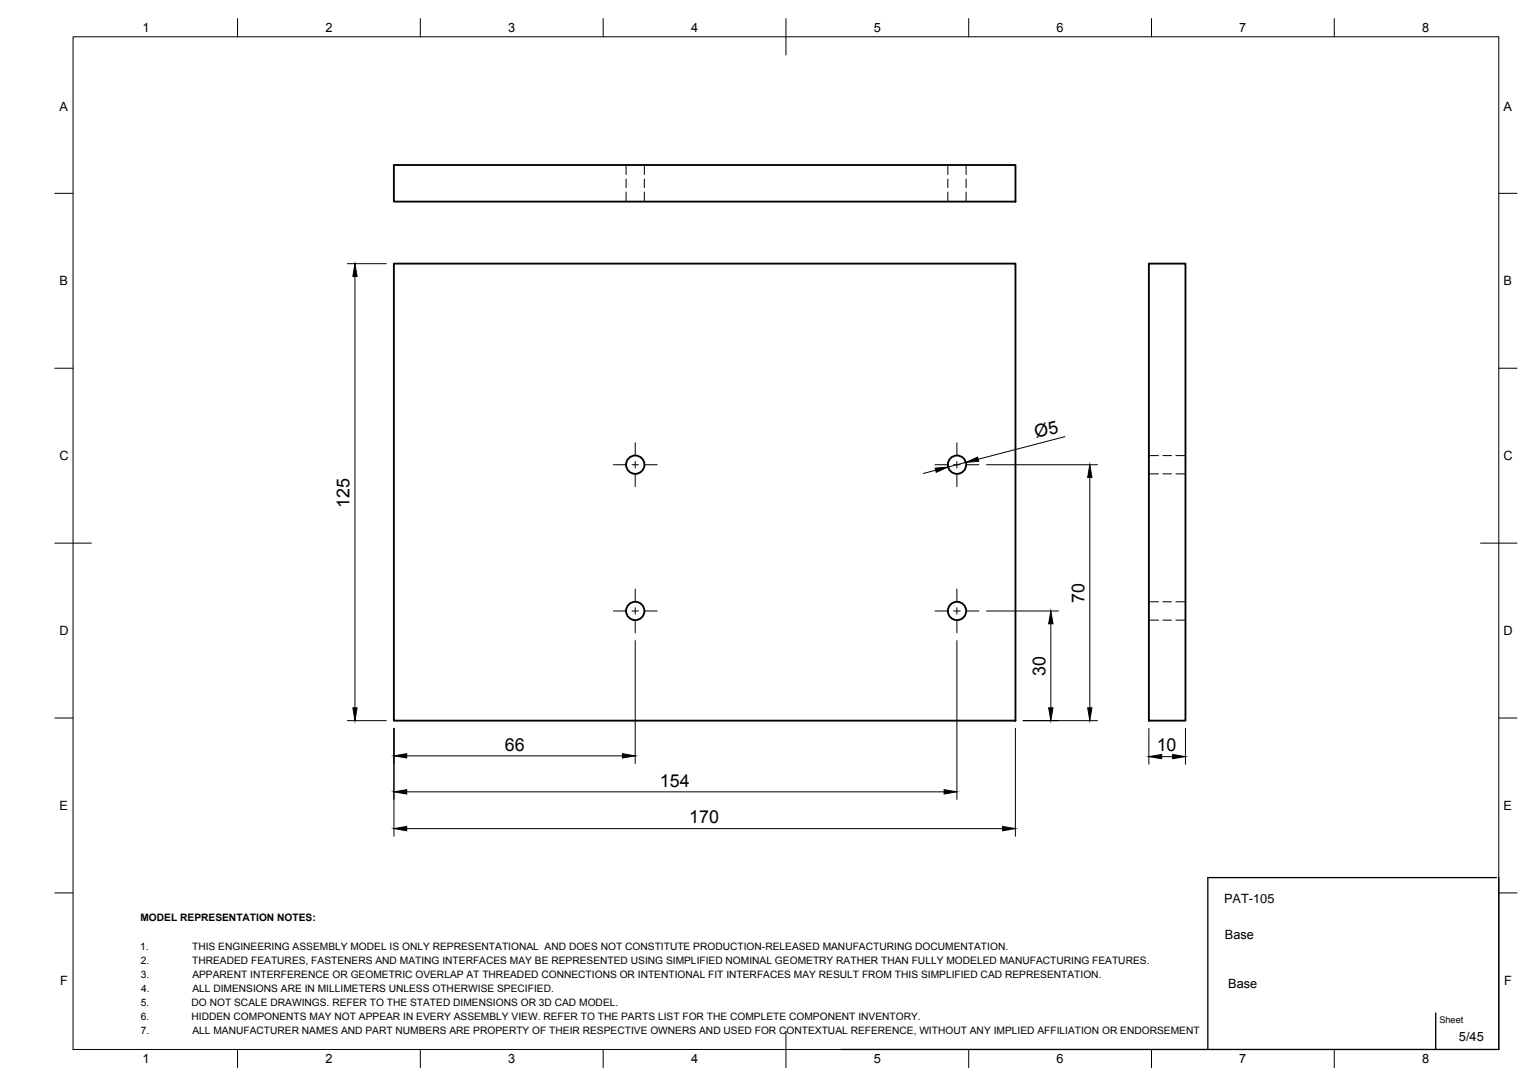
ISO-10303-21;
HEADER;
/* Generated by software containing ST-Developer
 * from STEP Tools, Inc. (www.steptools.com) 
 */

FILE_DESCRIPTION(
/* description */ ('Torque wrench calibration arm'),
/* implementation_level */ '2;1');

FILE_NAME(
/* name */ 'Base.step',
/* time_stamp */ '2026-10-28T03:24:52-07:00',
/* author */ (''),
/* organization */ (''),
/* preprocessor_version */ 'ST-DEVELOPER v20.2',
/* originating_system */ 'Autodesk Translation Framework v15.17.0.0',
/* authorisation */ '');

FILE_SCHEMA (('AUTOMOTIVE_DESIGN { 1 0 10303 214 3 1 1 }'));
ENDSEC;

DATA;
#10=MECHANICAL_DESIGN_GEOMETRIC_PRESENTATION_REPRESENTATION('',(#426),#12783);
#352=SHAPE_REPRESENTATION_RELATIONSHIP('SRR','None',#12933,#389);
#389=ADVANCED_BREP_SHAPE_REPRESENTATION('',(#480),#12742);
#426=STYLED_ITEM('',(#13191),#480);
#480=MANIFOLD_SOLID_BREP('Body1',#6495);
#531=FACE_BOUND('',#1279,.T.);
#532=FACE_BOUND('',#1280,.T.);
#533=FACE_BOUND('',#1281,.T.);
#534=FACE_BOUND('',#1282,.T.);
#535=FACE_BOUND('',#1284,.T.);
#536=FACE_BOUND('',#1285,.T.);
#537=FACE_BOUND('',#1286,.T.);
#538=FACE_BOUND('',#1287,.T.);
#652=PLANE('',#6975);
#653=PLANE('',#6976);
#654=PLANE('',#6977);
#655=PLANE('',#6978);
#656=PLANE('',#6979);
#657=PLANE('',#6980);
#875=FACE_OUTER_BOUND('',#1270,.T.);
#876=FACE_OUTER_BOUND('',#1271,.T.);
#877=FACE_OUTER_BOUND('',#1272,.T.);
#878=FACE_OUTER_BOUND('',#1273,.T.);
#879=FACE_OUTER_BOUND('',#1274,.T.);
#880=FACE_OUTER_BOUND('',#1275,.T.);
#881=FACE_OUTER_BOUND('',#1276,.T.);
#882=FACE_OUTER_BOUND('',#1277,.T.);
#883=FACE_OUTER_BOUND('',#1278,.T.);
#884=FACE_OUTER_BOUND('',#1283,.T.);
#1270=EDGE_LOOP('',(#4351,#4352,#4353,#4354));
#1271=EDGE_LOOP('',(#4355,#4356,#4357,#4358));
#1272=EDGE_LOOP('',(#4359,#4360,#4361,#4362));
#1273=EDGE_LOOP('',(#4363,#4364,#4365,#4366));
#1274=EDGE_LOOP('',(#4367,#4368,#4369,#4370));
#1275=EDGE_LOOP('',(#4371,#4372,#4373,#4374));
#1276=EDGE_LOOP('',(#4375,#4376,#4377,#4378));
#1277=EDGE_LOOP('',(#4379,#4380,#4381,#4382));
#1278=EDGE_LOOP('',(#4383,#4384,#4385,#4386));
#1279=EDGE_LOOP('',(#4387));
#1280=EDGE_LOOP('',(#4388));
#1281=EDGE_LOOP('',(#4389));
#1282=EDGE_LOOP('',(#4390));
#1283=EDGE_LOOP('',(#4391,#4392,#4393,#4394));
#1284=EDGE_LOOP('',(#4395));
#1285=EDGE_LOOP('',(#4396));
#1286=EDGE_LOOP('',(#4397));
#1287=EDGE_LOOP('',(#4398));
#1786=LINE('',#9932,#2201);
#1787=LINE('',#9938,#2202);
#1788=LINE('',#9944,#2203);
#1789=LINE('',#9950,#2204);
#1790=LINE('',#9955,#2205);
#1791=LINE('',#9957,#2206);
#1792=LINE('',#9959,#2207);
#1793=LINE('',#9960,#2208);
#1794=LINE('',#9963,#2209);
#1795=LINE('',#9965,#2210);
#1796=LINE('',#9966,#2211);
#1797=LINE('',#9969,#2212);
#1798=LINE('',#9971,#2213);
#1799=LINE('',#9972,#2214);
#1800=LINE('',#9974,#2215);
#1801=LINE('',#9975,#2216);
#2201=VECTOR('',#7820,0.25);
#2202=VECTOR('',#7827,0.25);
#2203=VECTOR('',#7834,0.25);
#2204=VECTOR('',#7841,0.25);
#2205=VECTOR('',#7846,1.);
#2206=VECTOR('',#7847,1.);
#2207=VECTOR('',#7848,1.);
#2208=VECTOR('',#7849,1.);
#2209=VECTOR('',#7852,1.);
#2210=VECTOR('',#7853,1.);
#2211=VECTOR('',#7854,1.);
#2212=VECTOR('',#7857,1.);
#2213=VECTOR('',#7858,1.);
#2214=VECTOR('',#7859,1.);
#2215=VECTOR('',#7862,1.);
#2216=VECTOR('',#7863,1.);
#2616=CIRCLE('',#6964,0.25);
#2617=CIRCLE('',#6965,0.25);
#2618=CIRCLE('',#6967,0.25);
#2619=CIRCLE('',#6968,0.25);
#2620=CIRCLE('',#6970,0.25);
#2621=CIRCLE('',#6971,0.25);
#2622=CIRCLE('',#6973,0.25);
#2623=CIRCLE('',#6974,0.25);
#2971=VERTEX_POINT('',#9929);
#2972=VERTEX_POINT('',#9931);
#2973=VERTEX_POINT('',#9935);
#2974=VERTEX_POINT('',#9937);
#2975=VERTEX_POINT('',#9941);
#2976=VERTEX_POINT('',#9943);
#2977=VERTEX_POINT('',#9947);
#2978=VERTEX_POINT('',#9949);
#2979=VERTEX_POINT('',#9953);
#2980=VERTEX_POINT('',#9954);
#2981=VERTEX_POINT('',#9956);
#2982=VERTEX_POINT('',#9958);
#2983=VERTEX_POINT('',#9962);
#2984=VERTEX_POINT('',#9964);
#2985=VERTEX_POINT('',#9968);
#2986=VERTEX_POINT('',#9970);
#3533=EDGE_CURVE('',#2971,#2971,#2616,.T.);
#3534=EDGE_CURVE('',#2971,#2972,#1786,.T.);
#3535=EDGE_CURVE('',#2972,#2972,#2617,.T.);
#3536=EDGE_CURVE('',#2973,#2973,#2618,.T.);
#3537=EDGE_CURVE('',#2973,#2974,#1787,.T.);
#3538=EDGE_CURVE('',#2974,#2974,#2619,.T.);
#3539=EDGE_CURVE('',#2975,#2975,#2620,.T.);
#3540=EDGE_CURVE('',#2975,#2976,#1788,.T.);
#3541=EDGE_CURVE('',#2976,#2976,#2621,.T.);
#3542=EDGE_CURVE('',#2977,#2977,#2622,.T.);
#3543=EDGE_CURVE('',#2977,#2978,#1789,.T.);
#3544=EDGE_CURVE('',#2978,#2978,#2623,.T.);
#3545=EDGE_CURVE('',#2979,#2980,#1790,.T.);
#3546=EDGE_CURVE('',#2980,#2981,#1791,.T.);
#3547=EDGE_CURVE('',#2982,#2981,#1792,.T.);
#3548=EDGE_CURVE('',#2979,#2982,#1793,.T.);
#3549=EDGE_CURVE('',#2983,#2979,#1794,.T.);
#3550=EDGE_CURVE('',#2984,#2982,#1795,.T.);
#3551=EDGE_CURVE('',#2983,#2984,#1796,.T.);
#3552=EDGE_CURVE('',#2985,#2983,#1797,.T.);
#3553=EDGE_CURVE('',#2986,#2984,#1798,.T.);
#3554=EDGE_CURVE('',#2985,#2986,#1799,.T.);
#3555=EDGE_CURVE('',#2980,#2985,#1800,.T.);
#3556=EDGE_CURVE('',#2981,#2986,#1801,.T.);
#4351=ORIENTED_EDGE('',*,*,#3533,.F.);
#4352=ORIENTED_EDGE('',*,*,#3534,.T.);
#4353=ORIENTED_EDGE('',*,*,#3535,.F.);
#4354=ORIENTED_EDGE('',*,*,#3534,.F.);
#4355=ORIENTED_EDGE('',*,*,#3536,.F.);
#4356=ORIENTED_EDGE('',*,*,#3537,.T.);
#4357=ORIENTED_EDGE('',*,*,#3538,.F.);
#4358=ORIENTED_EDGE('',*,*,#3537,.F.);
#4359=ORIENTED_EDGE('',*,*,#3539,.F.);
#4360=ORIENTED_EDGE('',*,*,#3540,.T.);
#4361=ORIENTED_EDGE('',*,*,#3541,.F.);
#4362=ORIENTED_EDGE('',*,*,#3540,.F.);
#4363=ORIENTED_EDGE('',*,*,#3542,.F.);
#4364=ORIENTED_EDGE('',*,*,#3543,.T.);
#4365=ORIENTED_EDGE('',*,*,#3544,.F.);
#4366=ORIENTED_EDGE('',*,*,#3543,.F.);
#4367=ORIENTED_EDGE('',*,*,#3545,.T.);
#4368=ORIENTED_EDGE('',*,*,#3546,.T.);
#4369=ORIENTED_EDGE('',*,*,#3547,.F.);
#4370=ORIENTED_EDGE('',*,*,#3548,.F.);
#4371=ORIENTED_EDGE('',*,*,#3549,.T.);
#4372=ORIENTED_EDGE('',*,*,#3548,.T.);
#4373=ORIENTED_EDGE('',*,*,#3550,.F.);
#4374=ORIENTED_EDGE('',*,*,#3551,.F.);
#4375=ORIENTED_EDGE('',*,*,#3552,.T.);
#4376=ORIENTED_EDGE('',*,*,#3551,.T.);
#4377=ORIENTED_EDGE('',*,*,#3553,.F.);
#4378=ORIENTED_EDGE('',*,*,#3554,.F.);
#4379=ORIENTED_EDGE('',*,*,#3555,.T.);
#4380=ORIENTED_EDGE('',*,*,#3554,.T.);
#4381=ORIENTED_EDGE('',*,*,#3556,.F.);
#4382=ORIENTED_EDGE('',*,*,#3546,.F.);
#4383=ORIENTED_EDGE('',*,*,#3556,.T.);
#4384=ORIENTED_EDGE('',*,*,#3553,.T.);
#4385=ORIENTED_EDGE('',*,*,#3550,.T.);
#4386=ORIENTED_EDGE('',*,*,#3547,.T.);
#4387=ORIENTED_EDGE('',*,*,#3535,.T.);
#4388=ORIENTED_EDGE('',*,*,#3538,.T.);
#4389=ORIENTED_EDGE('',*,*,#3541,.T.);
#4390=ORIENTED_EDGE('',*,*,#3544,.T.);
#4391=ORIENTED_EDGE('',*,*,#3555,.F.);
#4392=ORIENTED_EDGE('',*,*,#3545,.F.);
#4393=ORIENTED_EDGE('',*,*,#3549,.F.);
#4394=ORIENTED_EDGE('',*,*,#3552,.F.);
#4395=ORIENTED_EDGE('',*,*,#3533,.T.);
#4396=ORIENTED_EDGE('',*,*,#3536,.T.);
#4397=ORIENTED_EDGE('',*,*,#3539,.T.);
#4398=ORIENTED_EDGE('',*,*,#3542,.T.);
#5987=CYLINDRICAL_SURFACE('',#6963,0.25);
#5988=CYLINDRICAL_SURFACE('',#6966,0.25);
#5989=CYLINDRICAL_SURFACE('',#6969,0.25);
#5990=CYLINDRICAL_SURFACE('',#6972,0.25);
#6100=ADVANCED_FACE('',(#875),#5987,.F.);
#6101=ADVANCED_FACE('',(#876),#5988,.F.);
#6102=ADVANCED_FACE('',(#877),#5989,.F.);
#6103=ADVANCED_FACE('',(#878),#5990,.F.);
#6104=ADVANCED_FACE('',(#879),#652,.T.);
#6105=ADVANCED_FACE('',(#880),#653,.T.);
#6106=ADVANCED_FACE('',(#881),#654,.T.);
#6107=ADVANCED_FACE('',(#882),#655,.T.);
#6108=ADVANCED_FACE('',(#883,#531,#532,#533,#534),#656,.T.);
#6109=ADVANCED_FACE('',(#884,#535,#536,#537,#538),#657,.F.);
#6495=CLOSED_SHELL('',(#6100,#6101,#6102,#6103,#6104,#6105,#6106,#6107,
#6108,#6109));
#6962=AXIS2_PLACEMENT_3D('',#9927,#7814,#7815);
#6963=AXIS2_PLACEMENT_3D('',#9928,#7816,#7817);
#6964=AXIS2_PLACEMENT_3D('',#9930,#7818,#7819);
#6965=AXIS2_PLACEMENT_3D('',#9933,#7821,#7822);
#6966=AXIS2_PLACEMENT_3D('',#9934,#7823,#7824);
#6967=AXIS2_PLACEMENT_3D('',#9936,#7825,#7826);
#6968=AXIS2_PLACEMENT_3D('',#9939,#7828,#7829);
#6969=AXIS2_PLACEMENT_3D('',#9940,#7830,#7831);
#6970=AXIS2_PLACEMENT_3D('',#9942,#7832,#7833);
#6971=AXIS2_PLACEMENT_3D('',#9945,#7835,#7836);
#6972=AXIS2_PLACEMENT_3D('',#9946,#7837,#7838);
#6973=AXIS2_PLACEMENT_3D('',#9948,#7839,#7840);
#6974=AXIS2_PLACEMENT_3D('',#9951,#7842,#7843);
#6975=AXIS2_PLACEMENT_3D('',#9952,#7844,#7845);
#6976=AXIS2_PLACEMENT_3D('',#9961,#7850,#7851);
#6977=AXIS2_PLACEMENT_3D('',#9967,#7855,#7856);
#6978=AXIS2_PLACEMENT_3D('',#9973,#7860,#7861);
#6979=AXIS2_PLACEMENT_3D('',#9976,#7864,#7865);
#6980=AXIS2_PLACEMENT_3D('',#9977,#7866,#7867);
#7814=DIRECTION('axis',(0.,0.,1.));
#7815=DIRECTION('refdir',(1.,0.,0.));
#7816=DIRECTION('center_axis',(0.,0.,1.));
#7817=DIRECTION('ref_axis',(1.,0.,0.));
#7818=DIRECTION('center_axis',(0.,0.,1.));
#7819=DIRECTION('ref_axis',(1.,0.,0.));
#7820=DIRECTION('',(0.,0.,1.));
#7821=DIRECTION('center_axis',(0.,0.,-1.));
#7822=DIRECTION('ref_axis',(1.,0.,0.));
#7823=DIRECTION('center_axis',(0.,0.,1.));
#7824=DIRECTION('ref_axis',(1.,0.,0.));
#7825=DIRECTION('center_axis',(0.,0.,1.));
#7826=DIRECTION('ref_axis',(1.,0.,0.));
#7827=DIRECTION('',(0.,0.,1.));
#7828=DIRECTION('center_axis',(0.,0.,-1.));
#7829=DIRECTION('ref_axis',(1.,0.,0.));
#7830=DIRECTION('center_axis',(0.,0.,1.));
#7831=DIRECTION('ref_axis',(1.,0.,0.));
#7832=DIRECTION('center_axis',(0.,0.,1.));
#7833=DIRECTION('ref_axis',(1.,0.,0.));
#7834=DIRECTION('',(0.,0.,1.));
#7835=DIRECTION('center_axis',(0.,0.,-1.));
#7836=DIRECTION('ref_axis',(1.,0.,0.));
#7837=DIRECTION('center_axis',(0.,0.,1.));
#7838=DIRECTION('ref_axis',(1.,0.,0.));
#7839=DIRECTION('center_axis',(0.,0.,1.));
#7840=DIRECTION('ref_axis',(1.,0.,0.));
#7841=DIRECTION('',(0.,0.,1.));
#7842=DIRECTION('center_axis',(0.,0.,-1.));
#7843=DIRECTION('ref_axis',(1.,0.,0.));
#7844=DIRECTION('center_axis',(0.,1.,0.));
#7845=DIRECTION('ref_axis',(-1.,0.,0.));
#7846=DIRECTION('',(-1.,0.,0.));
#7847=DIRECTION('',(0.,0.,1.));
#7848=DIRECTION('',(-1.,0.,0.));
#7849=DIRECTION('',(0.,0.,1.));
#7850=DIRECTION('center_axis',(1.,0.,0.));
#7851=DIRECTION('ref_axis',(0.,1.,0.));
#7852=DIRECTION('',(0.,1.,0.));
#7853=DIRECTION('',(0.,1.,0.));
#7854=DIRECTION('',(0.,0.,1.));
#7855=DIRECTION('center_axis',(0.,-1.,0.));
#7856=DIRECTION('ref_axis',(1.,0.,0.));
#7857=DIRECTION('',(1.,0.,0.));
#7858=DIRECTION('',(1.,0.,0.));
#7859=DIRECTION('',(0.,0.,1.));
#7860=DIRECTION('center_axis',(-1.,0.,0.));
#7861=DIRECTION('ref_axis',(0.,-1.,0.));
#7862=DIRECTION('',(0.,-1.,0.));
#7863=DIRECTION('',(0.,-1.,0.));
#7864=DIRECTION('center_axis',(0.,0.,1.));
#7865=DIRECTION('ref_axis',(1.,0.,0.));
#7866=DIRECTION('center_axis',(0.,0.,1.));
#7867=DIRECTION('ref_axis',(1.,0.,0.));
#9927=CARTESIAN_POINT('',(0.,0.,0.));
#9928=CARTESIAN_POINT('Origin',(4.4,1.,-0.1));
#9929=CARTESIAN_POINT('',(4.15,1.,0.));
#9930=CARTESIAN_POINT('Origin',(4.4,1.,0.));
#9931=CARTESIAN_POINT('',(4.15,1.,1.));
#9932=CARTESIAN_POINT('',(4.15,1.,-0.1));
#9933=CARTESIAN_POINT('Origin',(4.4,1.,1.));
#9934=CARTESIAN_POINT('Origin',(-4.4,5.,-0.1));
#9935=CARTESIAN_POINT('',(-4.65,5.,0.));
#9936=CARTESIAN_POINT('Origin',(-4.4,5.,0.));
#9937=CARTESIAN_POINT('',(-4.65,5.,1.));
#9938=CARTESIAN_POINT('',(-4.65,5.,-0.1));
#9939=CARTESIAN_POINT('Origin',(-4.4,5.,1.));
#9940=CARTESIAN_POINT('Origin',(-4.4,1.,-0.1));
#9941=CARTESIAN_POINT('',(-4.65,1.,0.));
#9942=CARTESIAN_POINT('Origin',(-4.4,1.,0.));
#9943=CARTESIAN_POINT('',(-4.65,1.,1.));
#9944=CARTESIAN_POINT('',(-4.65,1.,-0.1));
#9945=CARTESIAN_POINT('Origin',(-4.4,1.,1.));
#9946=CARTESIAN_POINT('Origin',(4.4,5.,-0.1));
#9947=CARTESIAN_POINT('',(4.15,5.,0.));
#9948=CARTESIAN_POINT('Origin',(4.4,5.,0.));
#9949=CARTESIAN_POINT('',(4.15,5.,1.));
#9950=CARTESIAN_POINT('',(4.15,5.,-0.1));
#9951=CARTESIAN_POINT('Origin',(4.4,5.,1.));
#9952=CARTESIAN_POINT('Origin',(11.,10.5,0.));
#9953=CARTESIAN_POINT('',(11.,10.5,0.));
#9954=CARTESIAN_POINT('',(-6.,10.5,0.));
#9955=CARTESIAN_POINT('',(11.,10.5,0.));
#9956=CARTESIAN_POINT('',(-6.,10.5,1.));
#9957=CARTESIAN_POINT('',(-6.,10.5,0.));
#9958=CARTESIAN_POINT('',(11.,10.5,1.));
#9959=CARTESIAN_POINT('',(11.,10.5,1.));
#9960=CARTESIAN_POINT('',(11.,10.5,0.));
#9961=CARTESIAN_POINT('Origin',(11.,-2.,0.));
#9962=CARTESIAN_POINT('',(11.,-2.,0.));
#9963=CARTESIAN_POINT('',(11.,-2.,0.));
#9964=CARTESIAN_POINT('',(11.,-2.,1.));
#9965=CARTESIAN_POINT('',(11.,-2.,1.));
#9966=CARTESIAN_POINT('',(11.,-2.,0.));
#9967=CARTESIAN_POINT('Origin',(-6.,-2.,0.));
#9968=CARTESIAN_POINT('',(-6.,-2.,0.));
#9969=CARTESIAN_POINT('',(-6.,-2.,0.));
#9970=CARTESIAN_POINT('',(-6.,-2.,1.));
#9971=CARTESIAN_POINT('',(-6.,-2.,1.));
#9972=CARTESIAN_POINT('',(-6.,-2.,0.));
#9973=CARTESIAN_POINT('Origin',(-6.,10.5,0.));
#9974=CARTESIAN_POINT('',(-6.,10.5,0.));
#9975=CARTESIAN_POINT('',(-6.,10.5,1.));
#9976=CARTESIAN_POINT('Origin',(2.5,4.25,1.));
#9977=CARTESIAN_POINT('Origin',(2.5,4.25,0.));
#12698=UNCERTAINTY_MEASURE_WITH_UNIT(LENGTH_MEASURE(0.001),#12784,
'DISTANCE_ACCURACY_VALUE',
'Maximum model space distance between geometric entities at asserted c
onnectivities');
#12739=UNCERTAINTY_MEASURE_WITH_UNIT(LENGTH_MEASURE(0.001),#12784,
'DISTANCE_ACCURACY_VALUE',
'Maximum model space distance between geometric entities at asserted c
onnectivities');
#12742=(
GEOMETRIC_REPRESENTATION_CONTEXT(3)
GLOBAL_UNCERTAINTY_ASSIGNED_CONTEXT((#12698))
GLOBAL_UNIT_ASSIGNED_CONTEXT((#12784,#12786,#12787))
REPRESENTATION_CONTEXT('','3D')
);
#12783=(
GEOMETRIC_REPRESENTATION_CONTEXT(3)
GLOBAL_UNCERTAINTY_ASSIGNED_CONTEXT((#12739))
GLOBAL_UNIT_ASSIGNED_CONTEXT((#12784,#12786,#12787))
REPRESENTATION_CONTEXT('','3D')
);
#12784=(
LENGTH_UNIT()
NAMED_UNIT(*)
SI_UNIT(.CENTI.,.METRE.)
);
#12786=(
NAMED_UNIT(*)
PLANE_ANGLE_UNIT()
SI_UNIT($,.RADIAN.)
);
#12787=(
NAMED_UNIT(*)
SI_UNIT($,.STERADIAN.)
SOLID_ANGLE_UNIT()
);
#12790=SHAPE_DEFINITION_REPRESENTATION(#12833,#12933);
#12833=PRODUCT_DEFINITION_SHAPE('',$,#12977);
#12933=SHAPE_REPRESENTATION('',(#6962),#12742);
#12974=PRODUCT_DEFINITION_CONTEXT('part definition',#13105,'design');
#12977=PRODUCT_DEFINITION('Base','Base',#13020,#12974);
#13020=PRODUCT_DEFINITION_FORMATION('',$,#13109);
#13105=APPLICATION_CONTEXT(
'Core Data for Automotive Mechanical Design Process');
#13106=PRODUCT_CONTEXT('part definition',#13105,'mechanical');
#13109=PRODUCT('Base','Base','Base',(#13106));
#13185=COLOUR_RGB('Dark Blue',0.08,0.2,0.34);
#13186=FILL_AREA_STYLE_COLOUR('',#13185);
#13187=FILL_AREA_STYLE('',(#13186));
#13188=SURFACE_STYLE_FILL_AREA(#13187);
#13189=SURFACE_SIDE_STYLE('',(#13188));
#13190=SURFACE_STYLE_USAGE(.BOTH.,#13189);
#13191=PRESENTATION_STYLE_ASSIGNMENT((#13190));
ENDSEC;
END-ISO-10303-21;
